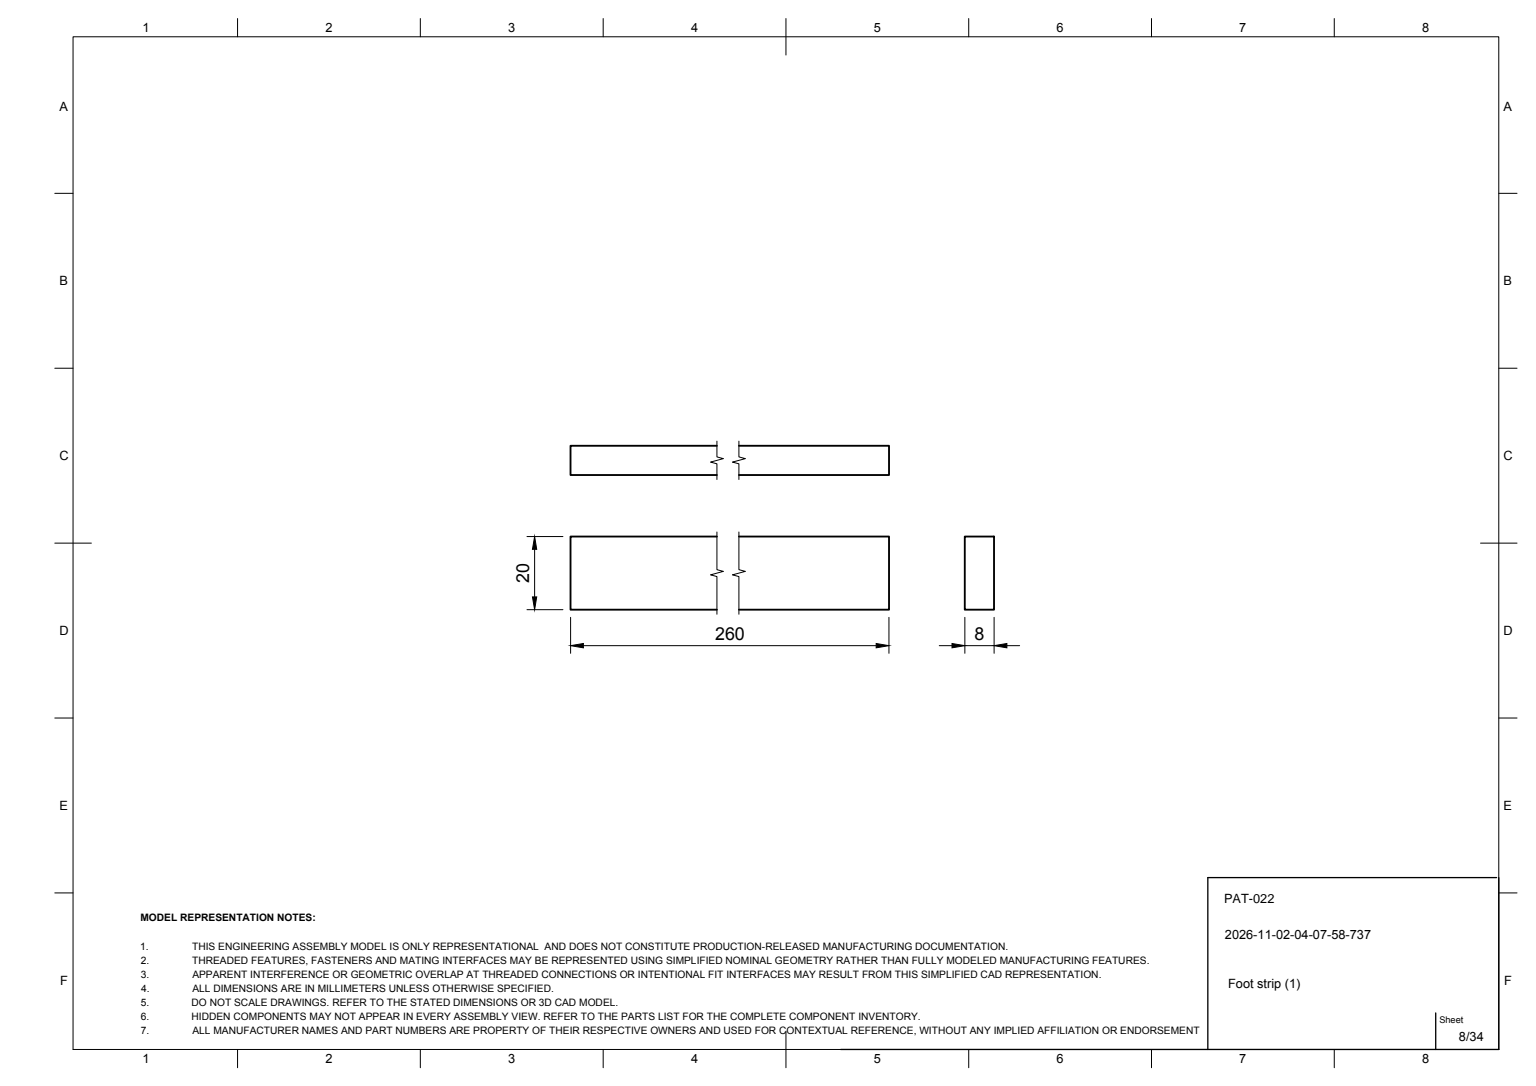
ISO-10303-21;
HEADER;
/* Generated by software containing ST-Developer
 * from STEP Tools, Inc. (www.steptools.com) 
 */

FILE_DESCRIPTION(
/* description */ ('Chute with adjustable gate'),
/* implementation_level */ '2;1');

FILE_NAME(
/* name */ 'Foot strip (1).step',
/* time_stamp */ '2026-10-27T10:52:28-07:00',
/* author */ (''),
/* organization */ (''),
/* preprocessor_version */ 'ST-DEVELOPER v20.2',
/* originating_system */ 'Autodesk Translation Framework v15.17.0.0',
/* authorisation */ '');

FILE_SCHEMA (('AUTOMOTIVE_DESIGN { 1 0 10303 214 3 1 1 }'));
ENDSEC;

DATA;
#10=MECHANICAL_DESIGN_GEOMETRIC_PRESENTATION_REPRESENTATION('',(#417),#13094);
#353=SHAPE_REPRESENTATION_RELATIONSHIP('SRR','None',#13254,#385);
#385=ADVANCED_BREP_SHAPE_REPRESENTATION('',(#449),#13063);
#417=STYLED_ITEM('',(#13481),#449);
#449=MANIFOLD_SOLID_BREP('Body1',#7600);
#612=PLANE('',#8038);
#613=PLANE('',#8039);
#614=PLANE('',#8040);
#615=PLANE('',#8041);
#616=PLANE('',#8042);
#617=PLANE('',#8043);
#944=FACE_OUTER_BOUND('',#1377,.T.);
#945=FACE_OUTER_BOUND('',#1378,.T.);
#946=FACE_OUTER_BOUND('',#1379,.T.);
#947=FACE_OUTER_BOUND('',#1380,.T.);
#948=FACE_OUTER_BOUND('',#1381,.T.);
#949=FACE_OUTER_BOUND('',#1382,.T.);
#1377=EDGE_LOOP('',(#5330,#5331,#5332,#5333));
#1378=EDGE_LOOP('',(#5334,#5335,#5336,#5337));
#1379=EDGE_LOOP('',(#5338,#5339,#5340,#5341));
#1380=EDGE_LOOP('',(#5342,#5343,#5344,#5345));
#1381=EDGE_LOOP('',(#5346,#5347,#5348,#5349));
#1382=EDGE_LOOP('',(#5350,#5351,#5352,#5353));
#1916=LINE('',#11058,#2693);
#1917=LINE('',#11060,#2694);
#1918=LINE('',#11062,#2695);
#1919=LINE('',#11063,#2696);
#1920=LINE('',#11066,#2697);
#1921=LINE('',#11068,#2698);
#1922=LINE('',#11069,#2699);
#1923=LINE('',#11072,#2700);
#1924=LINE('',#11074,#2701);
#1925=LINE('',#11075,#2702);
#1926=LINE('',#11077,#2703);
#1927=LINE('',#11078,#2704);
#2693=VECTOR('',#8860,1.);
#2694=VECTOR('',#8861,1.);
#2695=VECTOR('',#8862,1.);
#2696=VECTOR('',#8863,1.);
#2697=VECTOR('',#8866,1.);
#2698=VECTOR('',#8867,1.);
#2699=VECTOR('',#8868,1.);
#2700=VECTOR('',#8871,1.);
#2701=VECTOR('',#8872,1.);
#2702=VECTOR('',#8873,1.);
#2703=VECTOR('',#8876,1.);
#2704=VECTOR('',#8877,1.);
#3641=VERTEX_POINT('',#11056);
#3642=VERTEX_POINT('',#11057);
#3643=VERTEX_POINT('',#11059);
#3644=VERTEX_POINT('',#11061);
#3645=VERTEX_POINT('',#11065);
#3646=VERTEX_POINT('',#11067);
#3647=VERTEX_POINT('',#11071);
#3648=VERTEX_POINT('',#11073);
#4298=EDGE_CURVE('',#3641,#3642,#1916,.T.);
#4299=EDGE_CURVE('',#3642,#3643,#1917,.T.);
#4300=EDGE_CURVE('',#3644,#3643,#1918,.T.);
#4301=EDGE_CURVE('',#3641,#3644,#1919,.T.);
#4302=EDGE_CURVE('',#3645,#3641,#1920,.T.);
#4303=EDGE_CURVE('',#3646,#3644,#1921,.T.);
#4304=EDGE_CURVE('',#3645,#3646,#1922,.T.);
#4305=EDGE_CURVE('',#3647,#3645,#1923,.T.);
#4306=EDGE_CURVE('',#3648,#3646,#1924,.T.);
#4307=EDGE_CURVE('',#3647,#3648,#1925,.T.);
#4308=EDGE_CURVE('',#3642,#3647,#1926,.T.);
#4309=EDGE_CURVE('',#3643,#3648,#1927,.T.);
#5330=ORIENTED_EDGE('',*,*,#4298,.T.);
#5331=ORIENTED_EDGE('',*,*,#4299,.T.);
#5332=ORIENTED_EDGE('',*,*,#4300,.F.);
#5333=ORIENTED_EDGE('',*,*,#4301,.F.);
#5334=ORIENTED_EDGE('',*,*,#4302,.T.);
#5335=ORIENTED_EDGE('',*,*,#4301,.T.);
#5336=ORIENTED_EDGE('',*,*,#4303,.F.);
#5337=ORIENTED_EDGE('',*,*,#4304,.F.);
#5338=ORIENTED_EDGE('',*,*,#4305,.T.);
#5339=ORIENTED_EDGE('',*,*,#4304,.T.);
#5340=ORIENTED_EDGE('',*,*,#4306,.F.);
#5341=ORIENTED_EDGE('',*,*,#4307,.F.);
#5342=ORIENTED_EDGE('',*,*,#4308,.T.);
#5343=ORIENTED_EDGE('',*,*,#4307,.T.);
#5344=ORIENTED_EDGE('',*,*,#4309,.F.);
#5345=ORIENTED_EDGE('',*,*,#4299,.F.);
#5346=ORIENTED_EDGE('',*,*,#4309,.T.);
#5347=ORIENTED_EDGE('',*,*,#4306,.T.);
#5348=ORIENTED_EDGE('',*,*,#4303,.T.);
#5349=ORIENTED_EDGE('',*,*,#4300,.T.);
#5350=ORIENTED_EDGE('',*,*,#4308,.F.);
#5351=ORIENTED_EDGE('',*,*,#4298,.F.);
#5352=ORIENTED_EDGE('',*,*,#4302,.F.);
#5353=ORIENTED_EDGE('',*,*,#4305,.F.);
#7212=ADVANCED_FACE('',(#944),#612,.T.);
#7213=ADVANCED_FACE('',(#945),#613,.T.);
#7214=ADVANCED_FACE('',(#946),#614,.T.);
#7215=ADVANCED_FACE('',(#947),#615,.T.);
#7216=ADVANCED_FACE('',(#948),#616,.T.);
#7217=ADVANCED_FACE('',(#949),#617,.F.);
#7600=CLOSED_SHELL('',(#7212,#7213,#7214,#7215,#7216,#7217));
#8037=AXIS2_PLACEMENT_3D('',#11054,#8856,#8857);
#8038=AXIS2_PLACEMENT_3D('',#11055,#8858,#8859);
#8039=AXIS2_PLACEMENT_3D('',#11064,#8864,#8865);
#8040=AXIS2_PLACEMENT_3D('',#11070,#8869,#8870);
#8041=AXIS2_PLACEMENT_3D('',#11076,#8874,#8875);
#8042=AXIS2_PLACEMENT_3D('',#11079,#8878,#8879);
#8043=AXIS2_PLACEMENT_3D('',#11080,#8880,#8881);
#8856=DIRECTION('axis',(0.,0.,1.));
#8857=DIRECTION('refdir',(1.,0.,0.));
#8858=DIRECTION('center_axis',(0.,1.,0.));
#8859=DIRECTION('ref_axis',(-1.,0.,0.));
#8860=DIRECTION('',(-1.,0.,0.));
#8861=DIRECTION('',(0.,0.,1.));
#8862=DIRECTION('',(-1.,0.,0.));
#8863=DIRECTION('',(0.,0.,1.));
#8864=DIRECTION('center_axis',(1.,0.,0.));
#8865=DIRECTION('ref_axis',(0.,1.,0.));
#8866=DIRECTION('',(0.,1.,0.));
#8867=DIRECTION('',(0.,1.,0.));
#8868=DIRECTION('',(0.,0.,1.));
#8869=DIRECTION('center_axis',(0.,-1.,0.));
#8870=DIRECTION('ref_axis',(1.,0.,0.));
#8871=DIRECTION('',(1.,0.,0.));
#8872=DIRECTION('',(1.,0.,0.));
#8873=DIRECTION('',(0.,0.,1.));
#8874=DIRECTION('center_axis',(-1.,0.,0.));
#8875=DIRECTION('ref_axis',(0.,-1.,0.));
#8876=DIRECTION('',(0.,-1.,0.));
#8877=DIRECTION('',(0.,-1.,0.));
#8878=DIRECTION('center_axis',(0.,0.,1.));
#8879=DIRECTION('ref_axis',(1.,0.,0.));
#8880=DIRECTION('center_axis',(0.,0.,1.));
#8881=DIRECTION('ref_axis',(1.,0.,0.));
#11054=CARTESIAN_POINT('',(0.,0.,0.));
#11055=CARTESIAN_POINT('Origin',(26.,13.,-1.8));
#11056=CARTESIAN_POINT('',(26.,13.,-1.8));
#11057=CARTESIAN_POINT('',(24.,13.,-1.8));
#11058=CARTESIAN_POINT('',(26.,13.,-1.8));
#11059=CARTESIAN_POINT('',(24.,13.,-1.));
#11060=CARTESIAN_POINT('',(24.,13.,-1.8));
#11061=CARTESIAN_POINT('',(26.,13.,-1.));
#11062=CARTESIAN_POINT('',(26.,13.,-1.));
#11063=CARTESIAN_POINT('',(26.,13.,-1.8));
#11064=CARTESIAN_POINT('Origin',(26.,-13.,-1.8));
#11065=CARTESIAN_POINT('',(26.,-13.,-1.8));
#11066=CARTESIAN_POINT('',(26.,-13.,-1.8));
#11067=CARTESIAN_POINT('',(26.,-13.,-1.));
#11068=CARTESIAN_POINT('',(26.,-13.,-1.));
#11069=CARTESIAN_POINT('',(26.,-13.,-1.8));
#11070=CARTESIAN_POINT('Origin',(24.,-13.,-1.8));
#11071=CARTESIAN_POINT('',(24.,-13.,-1.8));
#11072=CARTESIAN_POINT('',(24.,-13.,-1.8));
#11073=CARTESIAN_POINT('',(24.,-13.,-1.));
#11074=CARTESIAN_POINT('',(24.,-13.,-1.));
#11075=CARTESIAN_POINT('',(24.,-13.,-1.8));
#11076=CARTESIAN_POINT('Origin',(24.,13.,-1.8));
#11077=CARTESIAN_POINT('',(24.,13.,-1.8));
#11078=CARTESIAN_POINT('',(24.,13.,-1.));
#11079=CARTESIAN_POINT('Origin',(25.,0.,-1.));
#11080=CARTESIAN_POINT('Origin',(25.,0.,-1.8));
#13026=UNCERTAINTY_MEASURE_WITH_UNIT(LENGTH_MEASURE(0.001),#13095,
'DISTANCE_ACCURACY_VALUE',
'Maximum model space distance between geometric entities at asserted c
onnectivities');
#13057=UNCERTAINTY_MEASURE_WITH_UNIT(LENGTH_MEASURE(0.001),#13095,
'DISTANCE_ACCURACY_VALUE',
'Maximum model space distance between geometric entities at asserted c
onnectivities');
#13063=(
GEOMETRIC_REPRESENTATION_CONTEXT(3)
GLOBAL_UNCERTAINTY_ASSIGNED_CONTEXT((#13026))
GLOBAL_UNIT_ASSIGNED_CONTEXT((#13095,#13097,#13098))
REPRESENTATION_CONTEXT('','3D')
);
#13094=(
GEOMETRIC_REPRESENTATION_CONTEXT(3)
GLOBAL_UNCERTAINTY_ASSIGNED_CONTEXT((#13057))
GLOBAL_UNIT_ASSIGNED_CONTEXT((#13095,#13097,#13098))
REPRESENTATION_CONTEXT('','3D')
);
#13095=(
LENGTH_UNIT()
NAMED_UNIT(*)
SI_UNIT(.CENTI.,.METRE.)
);
#13097=(
NAMED_UNIT(*)
PLANE_ANGLE_UNIT()
SI_UNIT($,.RADIAN.)
);
#13098=(
NAMED_UNIT(*)
SI_UNIT($,.STERADIAN.)
SOLID_ANGLE_UNIT()
);
#13104=SHAPE_DEFINITION_REPRESENTATION(#13140,#13254);
#13140=PRODUCT_DEFINITION_SHAPE('',$,#13291);
#13254=SHAPE_REPRESENTATION('',(#8037),#13063);
#13285=PRODUCT_DEFINITION_CONTEXT('part definition',#13395,'design');
#13291=PRODUCT_DEFINITION('Foot strip (1)','Foot strip (1)',#13327,#13285);
#13327=PRODUCT_DEFINITION_FORMATION('',$,#13402);
#13395=APPLICATION_CONTEXT(
'Core Data for Automotive Mechanical Design Process');
#13396=PRODUCT_CONTEXT('part definition',#13395,'mechanical');
#13402=PRODUCT('Foot strip (1)','Foot strip (1)','Foot strip (1)',(#13396));
#13475=COLOUR_RGB('Light Blue',0.38,0.62,0.78);
#13476=FILL_AREA_STYLE_COLOUR('',#13475);
#13477=FILL_AREA_STYLE('',(#13476));
#13478=SURFACE_STYLE_FILL_AREA(#13477);
#13479=SURFACE_SIDE_STYLE('',(#13478));
#13480=SURFACE_STYLE_USAGE(.BOTH.,#13479);
#13481=PRESENTATION_STYLE_ASSIGNMENT((#13480));
ENDSEC;
END-ISO-10303-21;
